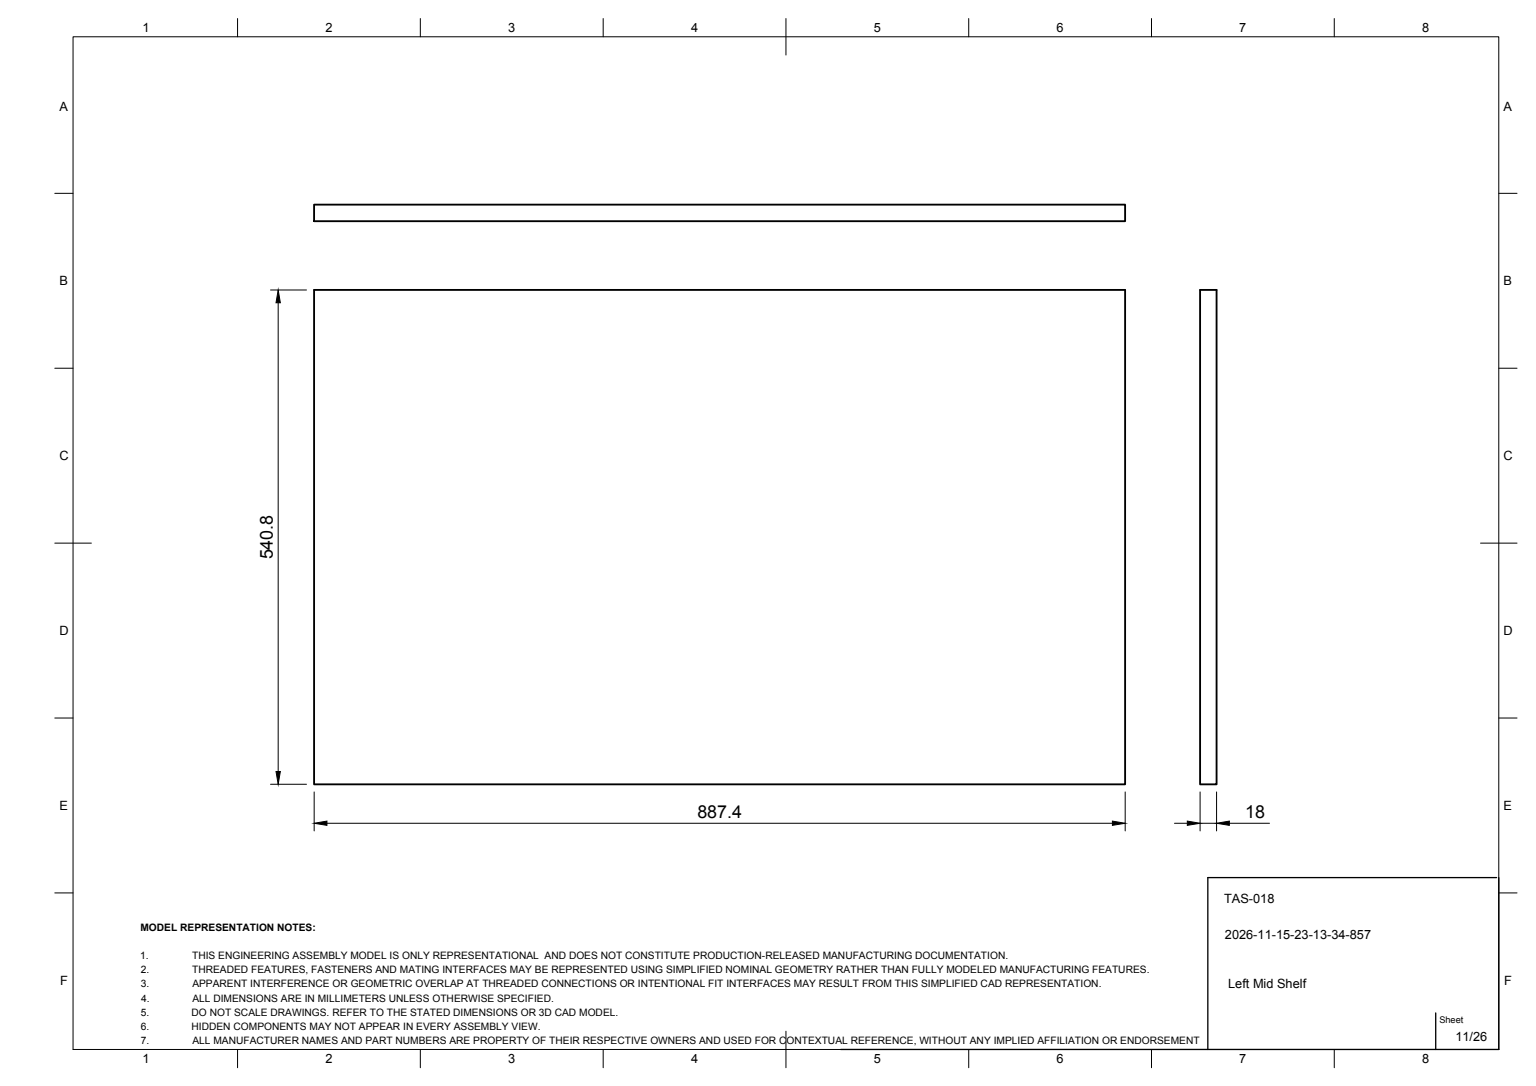
ISO-10303-21;
HEADER;
/* Generated by software containing ST-Developer
 * from STEP Tools, Inc. (www.steptools.com) 
 */

FILE_DESCRIPTION(
/* description */ (''),
/* implementation_level */ '2;1');

FILE_NAME(
/* name */ 'Left Mid Shelf.step',
/* time_stamp */ '2026-11-15T15:17:57-08:00',
/* author */ (''),
/* organization */ (''),
/* preprocessor_version */ 'ST-DEVELOPER v20.2',
/* originating_system */ 'Autodesk Translation Framework v15.17.0.0',
/* authorisation */ '');

FILE_SCHEMA (('AUTOMOTIVE_DESIGN { 1 0 10303 214 3 1 1 }'));
ENDSEC;

DATA;
#10=MECHANICAL_DESIGN_GEOMETRIC_PRESENTATION_REPRESENTATION('',(#186),#3723);
#138=SHAPE_REPRESENTATION_RELATIONSHIP('SRR','None',#3819,#162);
#162=ADVANCED_BREP_SHAPE_REPRESENTATION('',(#210),#3708);
#186=STYLED_ITEM('',(#3947),#210);
#210=MANIFOLD_SOLID_BREP('Body1',#2034);
#276=FACE_OUTER_BOUND('',#402,.T.);
#277=FACE_OUTER_BOUND('',#403,.T.);
#278=FACE_OUTER_BOUND('',#404,.T.);
#279=FACE_OUTER_BOUND('',#405,.T.);
#280=FACE_OUTER_BOUND('',#406,.T.);
#281=FACE_OUTER_BOUND('',#407,.T.);
#402=EDGE_LOOP('',(#1509,#1510,#1511,#1512));
#403=EDGE_LOOP('',(#1513,#1514,#1515,#1516));
#404=EDGE_LOOP('',(#1517,#1518,#1519,#1520));
#405=EDGE_LOOP('',(#1521,#1522,#1523,#1524));
#406=EDGE_LOOP('',(#1525,#1526,#1527,#1528));
#407=EDGE_LOOP('',(#1529,#1530,#1531,#1532));
#574=LINE('',#3335,#796);
#575=LINE('',#3337,#797);
#576=LINE('',#3339,#798);
#577=LINE('',#3340,#799);
#578=LINE('',#3344,#800);
#579=LINE('',#3346,#801);
#580=LINE('',#3348,#802);
#581=LINE('',#3349,#803);
#582=LINE('',#3351,#804);
#583=LINE('',#3352,#805);
#584=LINE('',#3354,#806);
#585=LINE('',#3356,#807);
#796=VECTOR('',#2734,34.9370078740157);
#797=VECTOR('',#2735,0.708661417322831);
#798=VECTOR('',#2736,34.9370078740157);
#799=VECTOR('',#2737,0.708661417322831);
#800=VECTOR('',#2740,0.708661417322831);
#801=VECTOR('',#2741,34.9370078740157);
#802=VECTOR('',#2742,0.708661417322831);
#803=VECTOR('',#2743,34.9370078740157);
#804=VECTOR('',#2746,21.2913385826772);
#805=VECTOR('',#2747,21.2913385826772);
#806=VECTOR('',#2750,21.2913385826772);
#807=VECTOR('',#2753,21.2913385826772);
#987=VERTEX_POINT('',#3333);
#988=VERTEX_POINT('',#3334);
#989=VERTEX_POINT('',#3336);
#990=VERTEX_POINT('',#3338);
#991=VERTEX_POINT('',#3342);
#992=VERTEX_POINT('',#3343);
#993=VERTEX_POINT('',#3345);
#994=VERTEX_POINT('',#3347);
#1176=EDGE_CURVE('',#987,#988,#574,.T.);
#1177=EDGE_CURVE('',#987,#989,#575,.T.);
#1178=EDGE_CURVE('',#989,#990,#576,.T.);
#1179=EDGE_CURVE('',#988,#990,#577,.T.);
#1180=EDGE_CURVE('',#991,#992,#578,.T.);
#1181=EDGE_CURVE('',#991,#993,#579,.T.);
#1182=EDGE_CURVE('',#993,#994,#580,.T.);
#1183=EDGE_CURVE('',#992,#994,#581,.T.);
#1184=EDGE_CURVE('',#987,#991,#582,.T.);
#1185=EDGE_CURVE('',#988,#993,#583,.T.);
#1186=EDGE_CURVE('',#990,#994,#584,.T.);
#1187=EDGE_CURVE('',#989,#992,#585,.T.);
#1509=ORIENTED_EDGE('',*,*,#1176,.F.);
#1510=ORIENTED_EDGE('',*,*,#1177,.T.);
#1511=ORIENTED_EDGE('',*,*,#1178,.T.);
#1512=ORIENTED_EDGE('',*,*,#1179,.F.);
#1513=ORIENTED_EDGE('',*,*,#1180,.F.);
#1514=ORIENTED_EDGE('',*,*,#1181,.T.);
#1515=ORIENTED_EDGE('',*,*,#1182,.T.);
#1516=ORIENTED_EDGE('',*,*,#1183,.F.);
#1517=ORIENTED_EDGE('',*,*,#1184,.F.);
#1518=ORIENTED_EDGE('',*,*,#1176,.T.);
#1519=ORIENTED_EDGE('',*,*,#1185,.T.);
#1520=ORIENTED_EDGE('',*,*,#1181,.F.);
#1521=ORIENTED_EDGE('',*,*,#1185,.F.);
#1522=ORIENTED_EDGE('',*,*,#1179,.T.);
#1523=ORIENTED_EDGE('',*,*,#1186,.T.);
#1524=ORIENTED_EDGE('',*,*,#1182,.F.);
#1525=ORIENTED_EDGE('',*,*,#1178,.F.);
#1526=ORIENTED_EDGE('',*,*,#1187,.T.);
#1527=ORIENTED_EDGE('',*,*,#1183,.T.);
#1528=ORIENTED_EDGE('',*,*,#1186,.F.);
#1529=ORIENTED_EDGE('',*,*,#1177,.F.);
#1530=ORIENTED_EDGE('',*,*,#1184,.T.);
#1531=ORIENTED_EDGE('',*,*,#1180,.T.);
#1532=ORIENTED_EDGE('',*,*,#1187,.F.);
#1829=PLANE('',#2380);
#1830=PLANE('',#2381);
#1831=PLANE('',#2382);
#1832=PLANE('',#2383);
#1833=PLANE('',#2384);
#1834=PLANE('',#2385);
#1950=ADVANCED_FACE('',(#276),#1829,.T.);
#1951=ADVANCED_FACE('',(#277),#1830,.F.);
#1952=ADVANCED_FACE('',(#278),#1831,.T.);
#1953=ADVANCED_FACE('',(#279),#1832,.T.);
#1954=ADVANCED_FACE('',(#280),#1833,.F.);
#1955=ADVANCED_FACE('',(#281),#1834,.F.);
#2034=CLOSED_SHELL('',(#1950,#1951,#1952,#1953,#1954,#1955));
#2379=AXIS2_PLACEMENT_3D('',#3331,#2730,#2731);
#2380=AXIS2_PLACEMENT_3D('',#3332,#2732,#2733);
#2381=AXIS2_PLACEMENT_3D('',#3341,#2738,#2739);
#2382=AXIS2_PLACEMENT_3D('',#3350,#2744,#2745);
#2383=AXIS2_PLACEMENT_3D('',#3353,#2748,#2749);
#2384=AXIS2_PLACEMENT_3D('',#3355,#2751,#2752);
#2385=AXIS2_PLACEMENT_3D('',#3357,#2754,#2755);
#2730=DIRECTION('axis',(0.,0.,1.));
#2731=DIRECTION('refdir',(1.,0.,0.));
#2732=DIRECTION('center_axis',(0.,0.,1.));
#2733=DIRECTION('ref_axis',(1.,0.,0.));
#2734=DIRECTION('',(1.,0.,0.));
#2735=DIRECTION('',(0.,-1.,0.));
#2736=DIRECTION('',(1.,0.,0.));
#2737=DIRECTION('',(0.,-1.,0.));
#2738=DIRECTION('center_axis',(0.,0.,1.));
#2739=DIRECTION('ref_axis',(1.,0.,0.));
#2740=DIRECTION('',(0.,-1.,0.));
#2741=DIRECTION('',(1.,0.,0.));
#2742=DIRECTION('',(0.,-1.,0.));
#2743=DIRECTION('',(1.,0.,0.));
#2744=DIRECTION('center_axis',(0.,1.,0.));
#2745=DIRECTION('ref_axis',(0.,0.,1.));
#2746=DIRECTION('',(0.,0.,-1.));
#2747=DIRECTION('',(0.,0.,-1.));
#2748=DIRECTION('center_axis',(1.,0.,0.));
#2749=DIRECTION('ref_axis',(0.,0.,-1.));
#2750=DIRECTION('',(0.,0.,-1.));
#2751=DIRECTION('center_axis',(0.,1.,0.));
#2752=DIRECTION('ref_axis',(0.,0.,1.));
#2753=DIRECTION('',(0.,0.,-1.));
#2754=DIRECTION('center_axis',(1.,0.,0.));
#2755=DIRECTION('ref_axis',(0.,0.,-1.));
#3331=CARTESIAN_POINT('',(0.,0.,0.));
#3332=CARTESIAN_POINT('Origin',(0.,0.,22.));
#3333=CARTESIAN_POINT('',(-35.2913385826772,25.,22.));
#3334=CARTESIAN_POINT('',(-0.354330708661419,25.,22.));
#3335=CARTESIAN_POINT('',(-35.2913385826772,25.,22.));
#3336=CARTESIAN_POINT('',(-35.2913385826772,24.2913385826772,22.));
#3337=CARTESIAN_POINT('',(-35.2913385826772,25.,22.));
#3338=CARTESIAN_POINT('',(-0.354330708661419,24.2913385826772,22.));
#3339=CARTESIAN_POINT('',(-35.2913385826772,24.2913385826772,22.));
#3340=CARTESIAN_POINT('',(-0.354330708661419,25.,22.));
#3341=CARTESIAN_POINT('Origin',(0.,0.,0.708661417322834));
#3342=CARTESIAN_POINT('',(-35.2913385826772,25.,0.708661417322834));
#3343=CARTESIAN_POINT('',(-35.2913385826772,24.2913385826772,0.708661417322834));
#3344=CARTESIAN_POINT('',(-35.2913385826772,25.,0.708661417322834));
#3345=CARTESIAN_POINT('',(-0.354330708661419,25.,0.708661417322834));
#3346=CARTESIAN_POINT('',(-35.2913385826772,25.,0.708661417322834));
#3347=CARTESIAN_POINT('',(-0.354330708661419,24.2913385826772,0.708661417322834));
#3348=CARTESIAN_POINT('',(-0.354330708661419,25.,0.708661417322834));
#3349=CARTESIAN_POINT('',(-35.2913385826772,24.2913385826772,0.708661417322834));
#3350=CARTESIAN_POINT('Origin',(-35.2913385826772,25.,56.9441943703592));
#3351=CARTESIAN_POINT('',(-35.2913385826772,25.,22.));
#3352=CARTESIAN_POINT('',(-0.354330708661419,25.,22.));
#3353=CARTESIAN_POINT('Origin',(-0.354330708661419,25.,56.9441943703592));
#3354=CARTESIAN_POINT('',(-0.354330708661419,24.2913385826772,22.));
#3355=CARTESIAN_POINT('Origin',(-35.2913385826772,24.2913385826772,56.9441943703592));
#3356=CARTESIAN_POINT('',(-35.2913385826772,24.2913385826772,22.));
#3357=CARTESIAN_POINT('Origin',(-35.2913385826772,25.,56.9441943703592));
#3681=UNCERTAINTY_MEASURE_WITH_UNIT(LENGTH_MEASURE(0.000393700787401575),
#3725,'DISTANCE_ACCURACY_VALUE',
'Maximum model space distance between geometric entities at asserted c
onnectivities');
#3696=UNCERTAINTY_MEASURE_WITH_UNIT(LENGTH_MEASURE(0.000393700787401575),
#3725,'DISTANCE_ACCURACY_VALUE',
'Maximum model space distance between geometric entities at asserted c
onnectivities');
#3708=(
GEOMETRIC_REPRESENTATION_CONTEXT(3)
GLOBAL_UNCERTAINTY_ASSIGNED_CONTEXT((#3681))
GLOBAL_UNIT_ASSIGNED_CONTEXT((#3725,#3729,#3730))
REPRESENTATION_CONTEXT('','3D')
);
#3723=(
GEOMETRIC_REPRESENTATION_CONTEXT(3)
GLOBAL_UNCERTAINTY_ASSIGNED_CONTEXT((#3696))
GLOBAL_UNIT_ASSIGNED_CONTEXT((#3725,#3729,#3730))
REPRESENTATION_CONTEXT('','3D')
);
#3724=DIMENSIONAL_EXPONENTS(1.,0.,0.,0.,0.,0.,0.);
#3725=(
CONVERSION_BASED_UNIT('inch',#3728)
LENGTH_UNIT()
NAMED_UNIT(#3724)
);
#3726=(
LENGTH_UNIT()
NAMED_UNIT(*)
SI_UNIT(.MILLI.,.METRE.)
);
#3728=LENGTH_MEASURE_WITH_UNIT(LENGTH_MEASURE(25.4),#3726);
#3729=(
NAMED_UNIT(*)
PLANE_ANGLE_UNIT()
SI_UNIT($,.RADIAN.)
);
#3730=(
NAMED_UNIT(*)
SI_UNIT($,.STERADIAN.)
SOLID_ANGLE_UNIT()
);
#3742=SHAPE_DEFINITION_REPRESENTATION(#3769,#3819);
#3769=PRODUCT_DEFINITION_SHAPE('',$,#3846);
#3819=SHAPE_REPRESENTATION('',(#2379),#3708);
#3834=PRODUCT_DEFINITION_CONTEXT('part definition',#3914,'design');
#3846=PRODUCT_DEFINITION('2026-11-15-23-13-34-857','Left Mid Shelf',#3872,
#3834);
#3872=PRODUCT_DEFINITION_FORMATION('',$,#3927);
#3914=APPLICATION_CONTEXT(
'Core Data for Automotive Mechanical Design Process');
#3915=PRODUCT_CONTEXT('part definition',#3914,'mechanical');
#3927=PRODUCT('2026-11-15-23-13-34-857','Left Mid Shelf',$,(#3915));
#3947=PRESENTATION_STYLE_ASSIGNMENT((#3955));
#3955=SURFACE_STYLE_USAGE(.BOTH.,#3963);
#3963=SURFACE_SIDE_STYLE('',(#3971));
#3971=SURFACE_STYLE_FILL_AREA(#3979);
#3979=FILL_AREA_STYLE('Light Blue',(#3987));
#3987=FILL_AREA_STYLE_COLOUR('Light Blue',#3995);
#3995=COLOUR_RGB('Light Blue',0.67843137254902,0.847058823529412,0.901960784313726);
ENDSEC;
END-ISO-10303-21;
